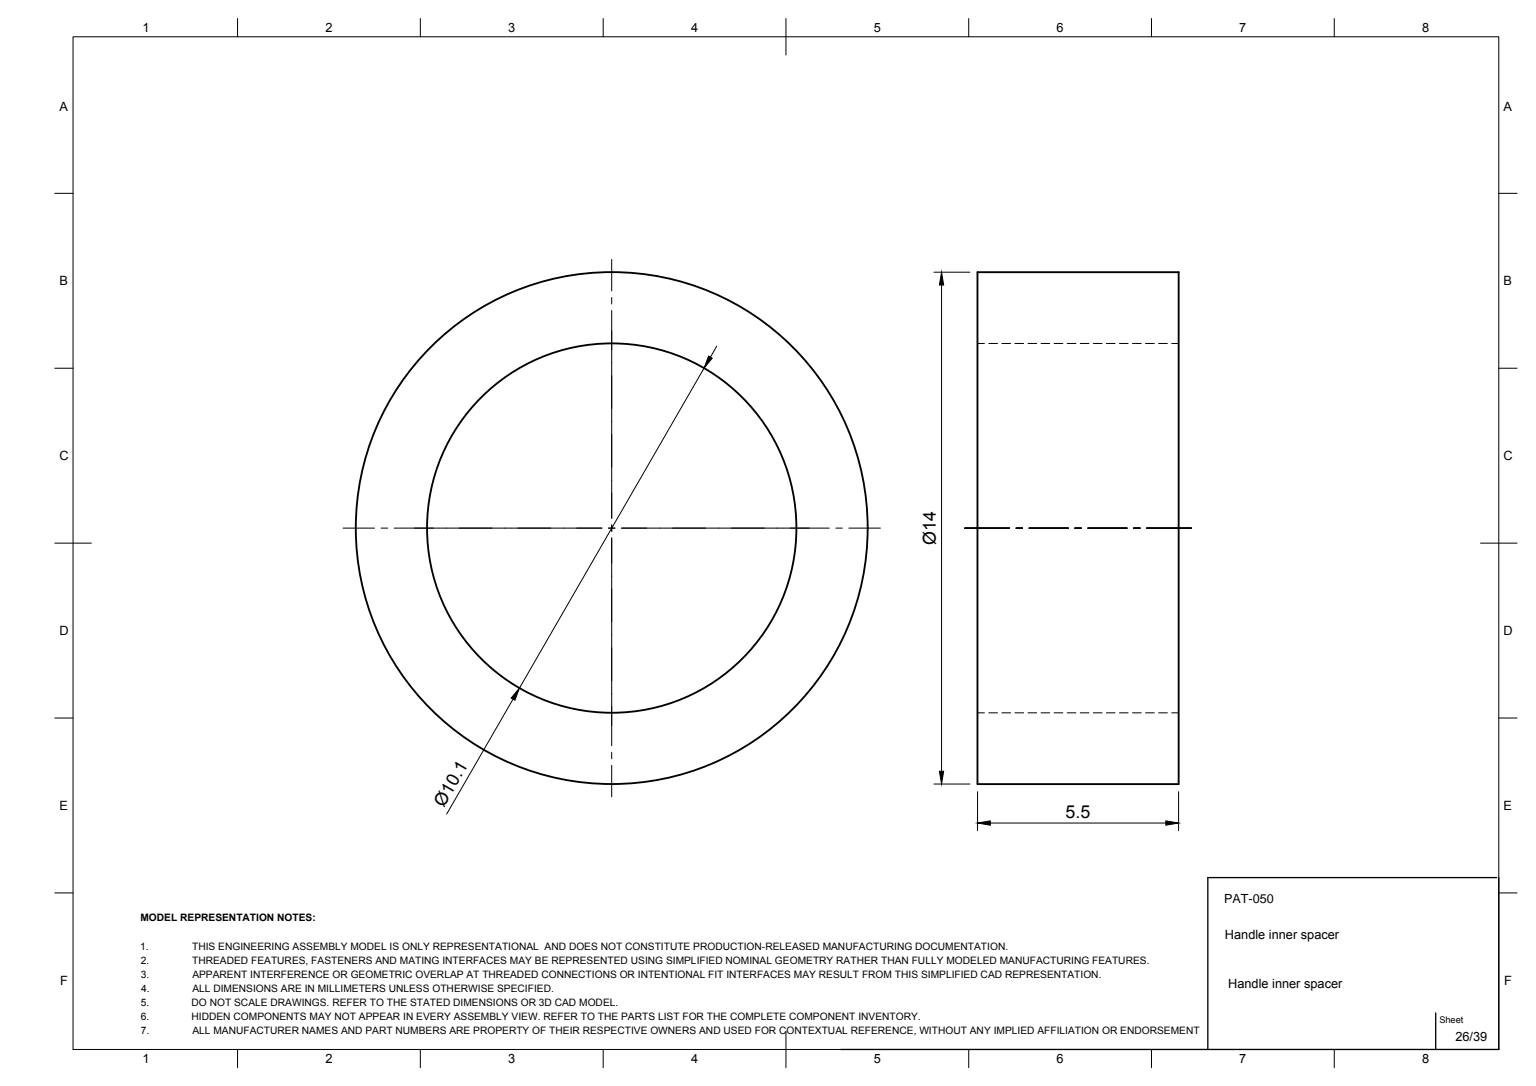
ISO-10303-21;
HEADER;
/* Generated by software containing ST-Developer
 * from STEP Tools, Inc. (www.steptools.com) 
 */

FILE_DESCRIPTION(
/* description */ ('Hand wheel with handle and shaft collar'),
/* implementation_level */ '2;1');

FILE_NAME(
/* name */ 'Handle inner spacer.step',
/* time_stamp */ '2026-10-28T03:23:19-07:00',
/* author */ (''),
/* organization */ (''),
/* preprocessor_version */ 'ST-DEVELOPER v20.2',
/* originating_system */ 'Autodesk Translation Framework v15.17.0.0',
/* authorisation */ '');

FILE_SCHEMA (('AUTOMOTIVE_DESIGN { 1 0 10303 214 3 1 1 }'));
ENDSEC;

DATA;
#10=MECHANICAL_DESIGN_GEOMETRIC_PRESENTATION_REPRESENTATION('',(#421),#10510);
#350=SHAPE_REPRESENTATION_RELATIONSHIP('SRR','None',#10668,#382);
#382=ADVANCED_BREP_SHAPE_REPRESENTATION('',(#467),#10495);
#421=STYLED_ITEM('',(#10894),#467);
#467=MANIFOLD_SOLID_BREP('Body1',#5321);
#577=FACE_BOUND('',#1367,.T.);
#578=FACE_BOUND('',#1369,.T.);
#698=PLANE('',#6117);
#699=PLANE('',#6118);
#954=FACE_OUTER_BOUND('',#1364,.T.);
#955=FACE_OUTER_BOUND('',#1365,.T.);
#956=FACE_OUTER_BOUND('',#1366,.T.);
#957=FACE_OUTER_BOUND('',#1368,.T.);
#1364=EDGE_LOOP('',(#4383,#4384,#4385,#4386));
#1365=EDGE_LOOP('',(#4387,#4388,#4389,#4390));
#1366=EDGE_LOOP('',(#4391));
#1367=EDGE_LOOP('',(#4392));
#1368=EDGE_LOOP('',(#4393));
#1369=EDGE_LOOP('',(#4394));
#1710=LINE('',#9491,#2020);
#1711=LINE('',#9497,#2021);
#2020=VECTOR('',#7448,0.505);
#2021=VECTOR('',#7455,0.7);
#2327=CIRCLE('',#6112,0.505);
#2328=CIRCLE('',#6113,0.505);
#2329=CIRCLE('',#6115,0.7);
#2330=CIRCLE('',#6116,0.7);
#2727=VERTEX_POINT('',#9488);
#2728=VERTEX_POINT('',#9490);
#2729=VERTEX_POINT('',#9494);
#2730=VERTEX_POINT('',#9496);
#3309=EDGE_CURVE('',#2727,#2727,#2327,.T.);
#3310=EDGE_CURVE('',#2727,#2728,#1710,.T.);
#3311=EDGE_CURVE('',#2728,#2728,#2328,.T.);
#3312=EDGE_CURVE('',#2729,#2729,#2329,.T.);
#3313=EDGE_CURVE('',#2729,#2730,#1711,.T.);
#3314=EDGE_CURVE('',#2730,#2730,#2330,.T.);
#4383=ORIENTED_EDGE('',*,*,#3309,.F.);
#4384=ORIENTED_EDGE('',*,*,#3310,.T.);
#4385=ORIENTED_EDGE('',*,*,#3311,.T.);
#4386=ORIENTED_EDGE('',*,*,#3310,.F.);
#4387=ORIENTED_EDGE('',*,*,#3312,.F.);
#4388=ORIENTED_EDGE('',*,*,#3313,.T.);
#4389=ORIENTED_EDGE('',*,*,#3314,.T.);
#4390=ORIENTED_EDGE('',*,*,#3313,.F.);
#4391=ORIENTED_EDGE('',*,*,#3312,.T.);
#4392=ORIENTED_EDGE('',*,*,#3309,.T.);
#4393=ORIENTED_EDGE('',*,*,#3314,.F.);
#4394=ORIENTED_EDGE('',*,*,#3311,.F.);
#4947=CYLINDRICAL_SURFACE('',#6111,0.505);
#4948=CYLINDRICAL_SURFACE('',#6114,0.7);
#5166=ADVANCED_FACE('',(#954),#4947,.F.);
#5167=ADVANCED_FACE('',(#955),#4948,.T.);
#5168=ADVANCED_FACE('',(#956,#577),#698,.T.);
#5169=ADVANCED_FACE('',(#957,#578),#699,.F.);
#5321=CLOSED_SHELL('',(#5166,#5167,#5168,#5169));
#6110=AXIS2_PLACEMENT_3D('',#9486,#7442,#7443);
#6111=AXIS2_PLACEMENT_3D('',#9487,#7444,#7445);
#6112=AXIS2_PLACEMENT_3D('',#9489,#7446,#7447);
#6113=AXIS2_PLACEMENT_3D('',#9492,#7449,#7450);
#6114=AXIS2_PLACEMENT_3D('',#9493,#7451,#7452);
#6115=AXIS2_PLACEMENT_3D('',#9495,#7453,#7454);
#6116=AXIS2_PLACEMENT_3D('',#9498,#7456,#7457);
#6117=AXIS2_PLACEMENT_3D('',#9499,#7458,#7459);
#6118=AXIS2_PLACEMENT_3D('',#9500,#7460,#7461);
#7442=DIRECTION('axis',(0.,0.,1.));
#7443=DIRECTION('refdir',(1.,0.,0.));
#7444=DIRECTION('center_axis',(0.,1.,0.));
#7445=DIRECTION('ref_axis',(1.,0.,0.));
#7446=DIRECTION('center_axis',(0.,-1.,0.));
#7447=DIRECTION('ref_axis',(1.,0.,0.));
#7448=DIRECTION('',(0.,-1.,0.));
#7449=DIRECTION('center_axis',(0.,-1.,0.));
#7450=DIRECTION('ref_axis',(1.,0.,0.));
#7451=DIRECTION('center_axis',(0.,1.,0.));
#7452=DIRECTION('ref_axis',(1.,0.,0.));
#7453=DIRECTION('center_axis',(0.,1.,0.));
#7454=DIRECTION('ref_axis',(1.,0.,0.));
#7455=DIRECTION('',(0.,-1.,0.));
#7456=DIRECTION('center_axis',(0.,1.,0.));
#7457=DIRECTION('ref_axis',(1.,0.,0.));
#7458=DIRECTION('center_axis',(0.,1.,0.));
#7459=DIRECTION('ref_axis',(1.,0.,0.));
#7460=DIRECTION('center_axis',(0.,1.,0.));
#7461=DIRECTION('ref_axis',(1.,0.,0.));
#9486=CARTESIAN_POINT('',(0.,0.,0.));
#9487=CARTESIAN_POINT('Origin',(6.5,-6.,10.));
#9488=CARTESIAN_POINT('',(5.995,-5.45,10.));
#9489=CARTESIAN_POINT('Origin',(6.5,-5.45,10.));
#9490=CARTESIAN_POINT('',(5.995,-6.,10.));
#9491=CARTESIAN_POINT('',(5.995,-6.,10.));
#9492=CARTESIAN_POINT('Origin',(6.5,-6.,10.));
#9493=CARTESIAN_POINT('Origin',(6.5,-6.,10.));
#9494=CARTESIAN_POINT('',(5.8,-5.45,10.));
#9495=CARTESIAN_POINT('Origin',(6.5,-5.45,10.));
#9496=CARTESIAN_POINT('',(5.8,-6.,10.));
#9497=CARTESIAN_POINT('',(5.8,-6.,10.));
#9498=CARTESIAN_POINT('Origin',(6.5,-6.,10.));
#9499=CARTESIAN_POINT('Origin',(6.5,-5.45,10.));
#9500=CARTESIAN_POINT('Origin',(6.5,-6.,10.));
#10456=UNCERTAINTY_MEASURE_WITH_UNIT(LENGTH_MEASURE(0.001),#10511,
'DISTANCE_ACCURACY_VALUE',
'Maximum model space distance between geometric entities at asserted c
onnectivities');
#10471=UNCERTAINTY_MEASURE_WITH_UNIT(LENGTH_MEASURE(0.001),#10511,
'DISTANCE_ACCURACY_VALUE',
'Maximum model space distance between geometric entities at asserted c
onnectivities');
#10495=(
GEOMETRIC_REPRESENTATION_CONTEXT(3)
GLOBAL_UNCERTAINTY_ASSIGNED_CONTEXT((#10456))
GLOBAL_UNIT_ASSIGNED_CONTEXT((#10511,#10513,#10514))
REPRESENTATION_CONTEXT('','3D')
);
#10510=(
GEOMETRIC_REPRESENTATION_CONTEXT(3)
GLOBAL_UNCERTAINTY_ASSIGNED_CONTEXT((#10471))
GLOBAL_UNIT_ASSIGNED_CONTEXT((#10511,#10513,#10514))
REPRESENTATION_CONTEXT('','3D')
);
#10511=(
LENGTH_UNIT()
NAMED_UNIT(*)
SI_UNIT(.CENTI.,.METRE.)
);
#10513=(
NAMED_UNIT(*)
PLANE_ANGLE_UNIT()
SI_UNIT($,.RADIAN.)
);
#10514=(
NAMED_UNIT(*)
SI_UNIT($,.STERADIAN.)
SOLID_ANGLE_UNIT()
);
#10538=SHAPE_DEFINITION_REPRESENTATION(#10581,#10668);
#10581=PRODUCT_DEFINITION_SHAPE('',$,#10707);
#10668=SHAPE_REPRESENTATION('',(#6110),#10495);
#10683=PRODUCT_DEFINITION_CONTEXT('part definition',#10799,'design');
#10707=PRODUCT_DEFINITION('Handle inner spacer','Handle inner spacer',#10745,
#10683);
#10745=PRODUCT_DEFINITION_FORMATION('',$,#10824);
#10799=APPLICATION_CONTEXT(
'Core Data for Automotive Mechanical Design Process');
#10800=PRODUCT_CONTEXT('part definition',#10799,'mechanical');
#10824=PRODUCT('Handle inner spacer','Handle inner spacer',
'Handle inner spacer',(#10800));
#10888=COLOUR_RGB('Light Blue',0.38,0.62,0.78);
#10889=FILL_AREA_STYLE_COLOUR('',#10888);
#10890=FILL_AREA_STYLE('',(#10889));
#10891=SURFACE_STYLE_FILL_AREA(#10890);
#10892=SURFACE_SIDE_STYLE('',(#10891));
#10893=SURFACE_STYLE_USAGE(.BOTH.,#10892);
#10894=PRESENTATION_STYLE_ASSIGNMENT((#10893));
ENDSEC;
END-ISO-10303-21;
